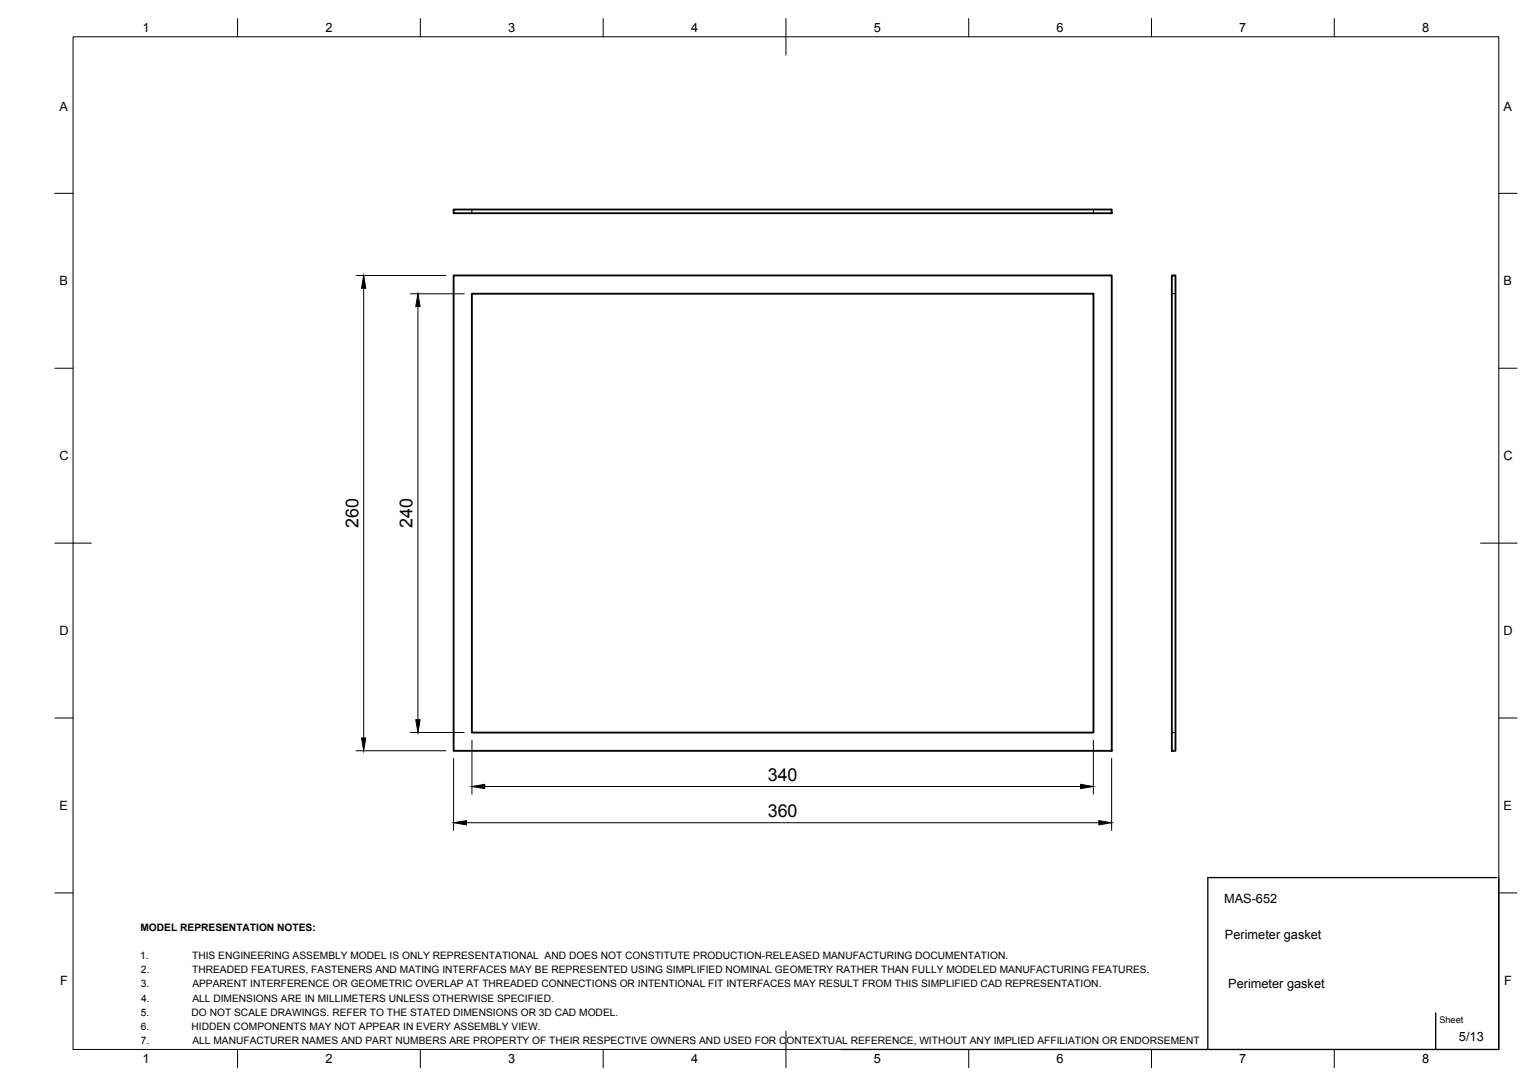
ISO-10303-21;
HEADER;
/* Generated by software containing ST-Developer
 * from STEP Tools, Inc. (www.steptools.com) 
 */

FILE_DESCRIPTION(
/* description */ ('Independent hinged machine back cover with retained hinge pins, perim
eter gasket and quarter-turn cam latch. Nominal cover 360 x 260 x 3 mm
, frame 430 x 300 x 20 mm. No guarding, structural or ingress rating a
ssigned.'),
/* implementation_level */ '2;1');

FILE_NAME(
/* name */ 'Perimeter gasket.step',
/* time_stamp */ '2026-11-09T19:36:59-08:00',
/* author */ (''),
/* organization */ (''),
/* preprocessor_version */ 'ST-DEVELOPER v20.2',
/* originating_system */ 'Autodesk Translation Framework v15.17.0.0',
/* authorisation */ '');

FILE_SCHEMA (('AUTOMOTIVE_DESIGN { 1 0 10303 214 3 1 1 }'));
ENDSEC;

DATA;
#10=MECHANICAL_DESIGN_GEOMETRIC_PRESENTATION_REPRESENTATION('',(#200),#32627);
#164=SHAPE_REPRESENTATION_RELATIONSHIP('SRR','None',#32710,#182);
#182=ADVANCED_BREP_SHAPE_REPRESENTATION('',(#218),#32611);
#200=STYLED_ITEM('',(#32809),#218);
#218=MANIFOLD_SOLID_BREP('Body1',#8677);
#250=FACE_BOUND('',#1133,.T.);
#251=FACE_BOUND('',#1135,.T.);
#335=PLANE('',#9103);
#336=PLANE('',#9104);
#337=PLANE('',#9105);
#338=PLANE('',#9106);
#339=PLANE('',#9107);
#340=PLANE('',#9108);
#341=PLANE('',#9109);
#342=PLANE('',#9110);
#343=PLANE('',#9111);
#344=PLANE('',#9112);
#633=FACE_OUTER_BOUND('',#1124,.T.);
#634=FACE_OUTER_BOUND('',#1125,.T.);
#635=FACE_OUTER_BOUND('',#1126,.T.);
#636=FACE_OUTER_BOUND('',#1127,.T.);
#637=FACE_OUTER_BOUND('',#1128,.T.);
#638=FACE_OUTER_BOUND('',#1129,.T.);
#639=FACE_OUTER_BOUND('',#1130,.T.);
#640=FACE_OUTER_BOUND('',#1131,.T.);
#641=FACE_OUTER_BOUND('',#1132,.T.);
#642=FACE_OUTER_BOUND('',#1134,.T.);
#1124=EDGE_LOOP('',(#6405,#6406,#6407,#6408));
#1125=EDGE_LOOP('',(#6409,#6410,#6411,#6412));
#1126=EDGE_LOOP('',(#6413,#6414,#6415,#6416));
#1127=EDGE_LOOP('',(#6417,#6418,#6419,#6420));
#1128=EDGE_LOOP('',(#6421,#6422,#6423,#6424));
#1129=EDGE_LOOP('',(#6425,#6426,#6427,#6428));
#1130=EDGE_LOOP('',(#6429,#6430,#6431,#6432));
#1131=EDGE_LOOP('',(#6433,#6434,#6435,#6436));
#1132=EDGE_LOOP('',(#6437,#6438,#6439,#6440));
#1133=EDGE_LOOP('',(#6441,#6442,#6443,#6444));
#1134=EDGE_LOOP('',(#6445,#6446,#6447,#6448));
#1135=EDGE_LOOP('',(#6449,#6450,#6451,#6452));
#2356=LINE('',#21698,#2902);
#2357=LINE('',#21700,#2903);
#2358=LINE('',#21702,#2904);
#2359=LINE('',#21703,#2905);
#2360=LINE('',#21706,#2906);
#2361=LINE('',#21708,#2907);
#2362=LINE('',#21709,#2908);
#2363=LINE('',#21712,#2909);
#2364=LINE('',#21714,#2910);
#2365=LINE('',#21715,#2911);
#2366=LINE('',#21717,#2912);
#2367=LINE('',#21718,#2913);
#2368=LINE('',#21722,#2914);
#2369=LINE('',#21724,#2915);
#2370=LINE('',#21726,#2916);
#2371=LINE('',#21727,#2917);
#2372=LINE('',#21730,#2918);
#2373=LINE('',#21732,#2919);
#2374=LINE('',#21733,#2920);
#2375=LINE('',#21736,#2921);
#2376=LINE('',#21738,#2922);
#2377=LINE('',#21739,#2923);
#2378=LINE('',#21741,#2924);
#2379=LINE('',#21742,#2925);
#2902=VECTOR('',#10134,10.);
#2903=VECTOR('',#10135,10.);
#2904=VECTOR('',#10136,10.);
#2905=VECTOR('',#10137,10.);
#2906=VECTOR('',#10140,10.);
#2907=VECTOR('',#10141,10.);
#2908=VECTOR('',#10142,10.);
#2909=VECTOR('',#10145,10.);
#2910=VECTOR('',#10146,10.);
#2911=VECTOR('',#10147,10.);
#2912=VECTOR('',#10150,10.);
#2913=VECTOR('',#10151,10.);
#2914=VECTOR('',#10154,10.);
#2915=VECTOR('',#10155,10.);
#2916=VECTOR('',#10156,10.);
#2917=VECTOR('',#10157,10.);
#2918=VECTOR('',#10160,10.);
#2919=VECTOR('',#10161,10.);
#2920=VECTOR('',#10162,10.);
#2921=VECTOR('',#10165,10.);
#2922=VECTOR('',#10166,10.);
#2923=VECTOR('',#10167,10.);
#2924=VECTOR('',#10170,10.);
#2925=VECTOR('',#10171,10.);
#3613=VERTEX_POINT('',#21696);
#3614=VERTEX_POINT('',#21697);
#3615=VERTEX_POINT('',#21699);
#3616=VERTEX_POINT('',#21701);
#3617=VERTEX_POINT('',#21705);
#3618=VERTEX_POINT('',#21707);
#3619=VERTEX_POINT('',#21711);
#3620=VERTEX_POINT('',#21713);
#3621=VERTEX_POINT('',#21720);
#3622=VERTEX_POINT('',#21721);
#3623=VERTEX_POINT('',#21723);
#3624=VERTEX_POINT('',#21725);
#3625=VERTEX_POINT('',#21729);
#3626=VERTEX_POINT('',#21731);
#3627=VERTEX_POINT('',#21735);
#3628=VERTEX_POINT('',#21737);
#4626=EDGE_CURVE('',#3613,#3614,#2356,.T.);
#4627=EDGE_CURVE('',#3614,#3615,#2357,.T.);
#4628=EDGE_CURVE('',#3616,#3615,#2358,.T.);
#4629=EDGE_CURVE('',#3613,#3616,#2359,.T.);
#4630=EDGE_CURVE('',#3617,#3613,#2360,.T.);
#4631=EDGE_CURVE('',#3618,#3616,#2361,.T.);
#4632=EDGE_CURVE('',#3617,#3618,#2362,.T.);
#4633=EDGE_CURVE('',#3619,#3617,#2363,.T.);
#4634=EDGE_CURVE('',#3620,#3618,#2364,.T.);
#4635=EDGE_CURVE('',#3619,#3620,#2365,.T.);
#4636=EDGE_CURVE('',#3614,#3619,#2366,.T.);
#4637=EDGE_CURVE('',#3615,#3620,#2367,.T.);
#4638=EDGE_CURVE('',#3621,#3622,#2368,.T.);
#4639=EDGE_CURVE('',#3622,#3623,#2369,.T.);
#4640=EDGE_CURVE('',#3624,#3623,#2370,.T.);
#4641=EDGE_CURVE('',#3621,#3624,#2371,.T.);
#4642=EDGE_CURVE('',#3625,#3621,#2372,.T.);
#4643=EDGE_CURVE('',#3626,#3624,#2373,.T.);
#4644=EDGE_CURVE('',#3625,#3626,#2374,.T.);
#4645=EDGE_CURVE('',#3627,#3625,#2375,.T.);
#4646=EDGE_CURVE('',#3628,#3626,#2376,.T.);
#4647=EDGE_CURVE('',#3627,#3628,#2377,.T.);
#4648=EDGE_CURVE('',#3622,#3627,#2378,.T.);
#4649=EDGE_CURVE('',#3623,#3628,#2379,.T.);
#6405=ORIENTED_EDGE('',*,*,#4626,.T.);
#6406=ORIENTED_EDGE('',*,*,#4627,.T.);
#6407=ORIENTED_EDGE('',*,*,#4628,.F.);
#6408=ORIENTED_EDGE('',*,*,#4629,.F.);
#6409=ORIENTED_EDGE('',*,*,#4630,.T.);
#6410=ORIENTED_EDGE('',*,*,#4629,.T.);
#6411=ORIENTED_EDGE('',*,*,#4631,.F.);
#6412=ORIENTED_EDGE('',*,*,#4632,.F.);
#6413=ORIENTED_EDGE('',*,*,#4633,.T.);
#6414=ORIENTED_EDGE('',*,*,#4632,.T.);
#6415=ORIENTED_EDGE('',*,*,#4634,.F.);
#6416=ORIENTED_EDGE('',*,*,#4635,.F.);
#6417=ORIENTED_EDGE('',*,*,#4636,.T.);
#6418=ORIENTED_EDGE('',*,*,#4635,.T.);
#6419=ORIENTED_EDGE('',*,*,#4637,.F.);
#6420=ORIENTED_EDGE('',*,*,#4627,.F.);
#6421=ORIENTED_EDGE('',*,*,#4638,.T.);
#6422=ORIENTED_EDGE('',*,*,#4639,.T.);
#6423=ORIENTED_EDGE('',*,*,#4640,.F.);
#6424=ORIENTED_EDGE('',*,*,#4641,.F.);
#6425=ORIENTED_EDGE('',*,*,#4642,.T.);
#6426=ORIENTED_EDGE('',*,*,#4641,.T.);
#6427=ORIENTED_EDGE('',*,*,#4643,.F.);
#6428=ORIENTED_EDGE('',*,*,#4644,.F.);
#6429=ORIENTED_EDGE('',*,*,#4645,.T.);
#6430=ORIENTED_EDGE('',*,*,#4644,.T.);
#6431=ORIENTED_EDGE('',*,*,#4646,.F.);
#6432=ORIENTED_EDGE('',*,*,#4647,.F.);
#6433=ORIENTED_EDGE('',*,*,#4648,.T.);
#6434=ORIENTED_EDGE('',*,*,#4647,.T.);
#6435=ORIENTED_EDGE('',*,*,#4649,.F.);
#6436=ORIENTED_EDGE('',*,*,#4639,.F.);
#6437=ORIENTED_EDGE('',*,*,#4649,.T.);
#6438=ORIENTED_EDGE('',*,*,#4646,.T.);
#6439=ORIENTED_EDGE('',*,*,#4643,.T.);
#6440=ORIENTED_EDGE('',*,*,#4640,.T.);
#6441=ORIENTED_EDGE('',*,*,#4637,.T.);
#6442=ORIENTED_EDGE('',*,*,#4634,.T.);
#6443=ORIENTED_EDGE('',*,*,#4631,.T.);
#6444=ORIENTED_EDGE('',*,*,#4628,.T.);
#6445=ORIENTED_EDGE('',*,*,#4648,.F.);
#6446=ORIENTED_EDGE('',*,*,#4638,.F.);
#6447=ORIENTED_EDGE('',*,*,#4642,.F.);
#6448=ORIENTED_EDGE('',*,*,#4645,.F.);
#6449=ORIENTED_EDGE('',*,*,#4636,.F.);
#6450=ORIENTED_EDGE('',*,*,#4626,.F.);
#6451=ORIENTED_EDGE('',*,*,#4630,.F.);
#6452=ORIENTED_EDGE('',*,*,#4633,.F.);
#8381=ADVANCED_FACE('',(#633),#335,.T.);
#8382=ADVANCED_FACE('',(#634),#336,.T.);
#8383=ADVANCED_FACE('',(#635),#337,.T.);
#8384=ADVANCED_FACE('',(#636),#338,.T.);
#8385=ADVANCED_FACE('',(#637),#339,.T.);
#8386=ADVANCED_FACE('',(#638),#340,.T.);
#8387=ADVANCED_FACE('',(#639),#341,.T.);
#8388=ADVANCED_FACE('',(#640),#342,.T.);
#8389=ADVANCED_FACE('',(#641,#250),#343,.T.);
#8390=ADVANCED_FACE('',(#642,#251),#344,.F.);
#8677=CLOSED_SHELL('',(#8381,#8382,#8383,#8384,#8385,#8386,#8387,#8388,
#8389,#8390));
#9102=AXIS2_PLACEMENT_3D('',#21694,#10130,#10131);
#9103=AXIS2_PLACEMENT_3D('',#21695,#10132,#10133);
#9104=AXIS2_PLACEMENT_3D('',#21704,#10138,#10139);
#9105=AXIS2_PLACEMENT_3D('',#21710,#10143,#10144);
#9106=AXIS2_PLACEMENT_3D('',#21716,#10148,#10149);
#9107=AXIS2_PLACEMENT_3D('',#21719,#10152,#10153);
#9108=AXIS2_PLACEMENT_3D('',#21728,#10158,#10159);
#9109=AXIS2_PLACEMENT_3D('',#21734,#10163,#10164);
#9110=AXIS2_PLACEMENT_3D('',#21740,#10168,#10169);
#9111=AXIS2_PLACEMENT_3D('',#21743,#10172,#10173);
#9112=AXIS2_PLACEMENT_3D('',#21744,#10174,#10175);
#10130=DIRECTION('axis',(0.,0.,1.));
#10131=DIRECTION('refdir',(1.,0.,0.));
#10132=DIRECTION('center_axis',(0.,1.,0.));
#10133=DIRECTION('ref_axis',(-1.,0.,0.));
#10134=DIRECTION('',(-1.,0.,0.));
#10135=DIRECTION('',(0.,0.,1.));
#10136=DIRECTION('',(-1.,0.,0.));
#10137=DIRECTION('',(0.,0.,1.));
#10138=DIRECTION('center_axis',(-1.,0.,0.));
#10139=DIRECTION('ref_axis',(0.,-1.,0.));
#10140=DIRECTION('',(0.,-1.,0.));
#10141=DIRECTION('',(0.,-1.,0.));
#10142=DIRECTION('',(0.,0.,1.));
#10143=DIRECTION('center_axis',(0.,-1.,0.));
#10144=DIRECTION('ref_axis',(1.,0.,0.));
#10145=DIRECTION('',(1.,0.,0.));
#10146=DIRECTION('',(1.,0.,0.));
#10147=DIRECTION('',(0.,0.,1.));
#10148=DIRECTION('center_axis',(1.,0.,0.));
#10149=DIRECTION('ref_axis',(0.,1.,0.));
#10150=DIRECTION('',(0.,1.,0.));
#10151=DIRECTION('',(0.,1.,0.));
#10152=DIRECTION('center_axis',(0.,1.,0.));
#10153=DIRECTION('ref_axis',(-1.,0.,0.));
#10154=DIRECTION('',(-1.,0.,0.));
#10155=DIRECTION('',(0.,0.,1.));
#10156=DIRECTION('',(-1.,0.,0.));
#10157=DIRECTION('',(0.,0.,1.));
#10158=DIRECTION('center_axis',(1.,0.,0.));
#10159=DIRECTION('ref_axis',(0.,1.,0.));
#10160=DIRECTION('',(0.,1.,0.));
#10161=DIRECTION('',(0.,1.,0.));
#10162=DIRECTION('',(0.,0.,1.));
#10163=DIRECTION('center_axis',(0.,-1.,0.));
#10164=DIRECTION('ref_axis',(1.,0.,0.));
#10165=DIRECTION('',(1.,0.,0.));
#10166=DIRECTION('',(1.,0.,0.));
#10167=DIRECTION('',(0.,0.,1.));
#10168=DIRECTION('center_axis',(-1.,0.,0.));
#10169=DIRECTION('ref_axis',(0.,-1.,0.));
#10170=DIRECTION('',(0.,-1.,0.));
#10171=DIRECTION('',(0.,-1.,0.));
#10172=DIRECTION('center_axis',(0.,0.,1.));
#10173=DIRECTION('ref_axis',(1.,0.,0.));
#10174=DIRECTION('center_axis',(0.,0.,1.));
#10175=DIRECTION('ref_axis',(1.,0.,0.));
#21694=CARTESIAN_POINT('',(0.,0.,0.));
#21695=CARTESIAN_POINT('Origin',(170.,-120.,0.));
#21696=CARTESIAN_POINT('',(170.,-120.,0.));
#21697=CARTESIAN_POINT('',(-170.,-120.,0.));
#21698=CARTESIAN_POINT('',(-170.,-120.,0.));
#21699=CARTESIAN_POINT('',(-170.,-120.,2.));
#21700=CARTESIAN_POINT('',(-170.,-120.,0.));
#21701=CARTESIAN_POINT('',(170.,-120.,2.));
#21702=CARTESIAN_POINT('',(-170.,-120.,2.));
#21703=CARTESIAN_POINT('',(170.,-120.,0.));
#21704=CARTESIAN_POINT('Origin',(170.,120.,0.));
#21705=CARTESIAN_POINT('',(170.,120.,0.));
#21706=CARTESIAN_POINT('',(170.,-120.,0.));
#21707=CARTESIAN_POINT('',(170.,120.,2.));
#21708=CARTESIAN_POINT('',(170.,-120.,2.));
#21709=CARTESIAN_POINT('',(170.,120.,0.));
#21710=CARTESIAN_POINT('Origin',(-170.,120.,0.));
#21711=CARTESIAN_POINT('',(-170.,120.,0.));
#21712=CARTESIAN_POINT('',(170.,120.,0.));
#21713=CARTESIAN_POINT('',(-170.,120.,2.));
#21714=CARTESIAN_POINT('',(170.,120.,2.));
#21715=CARTESIAN_POINT('',(-170.,120.,0.));
#21716=CARTESIAN_POINT('Origin',(-170.,-120.,0.));
#21717=CARTESIAN_POINT('',(-170.,120.,0.));
#21718=CARTESIAN_POINT('',(-170.,120.,2.));
#21719=CARTESIAN_POINT('Origin',(180.,130.,0.));
#21720=CARTESIAN_POINT('',(180.,130.,0.));
#21721=CARTESIAN_POINT('',(-180.,130.,0.));
#21722=CARTESIAN_POINT('',(180.,130.,0.));
#21723=CARTESIAN_POINT('',(-180.,130.,2.));
#21724=CARTESIAN_POINT('',(-180.,130.,0.));
#21725=CARTESIAN_POINT('',(180.,130.,2.));
#21726=CARTESIAN_POINT('',(180.,130.,2.));
#21727=CARTESIAN_POINT('',(180.,130.,0.));
#21728=CARTESIAN_POINT('Origin',(180.,-130.,0.));
#21729=CARTESIAN_POINT('',(180.,-130.,0.));
#21730=CARTESIAN_POINT('',(180.,-130.,0.));
#21731=CARTESIAN_POINT('',(180.,-130.,2.));
#21732=CARTESIAN_POINT('',(180.,-130.,2.));
#21733=CARTESIAN_POINT('',(180.,-130.,0.));
#21734=CARTESIAN_POINT('Origin',(-180.,-130.,0.));
#21735=CARTESIAN_POINT('',(-180.,-130.,0.));
#21736=CARTESIAN_POINT('',(-180.,-130.,0.));
#21737=CARTESIAN_POINT('',(-180.,-130.,2.));
#21738=CARTESIAN_POINT('',(-180.,-130.,2.));
#21739=CARTESIAN_POINT('',(-180.,-130.,0.));
#21740=CARTESIAN_POINT('Origin',(-180.,130.,0.));
#21741=CARTESIAN_POINT('',(-180.,130.,0.));
#21742=CARTESIAN_POINT('',(-180.,130.,2.));
#21743=CARTESIAN_POINT('Origin',(0.,0.,2.));
#21744=CARTESIAN_POINT('Origin',(0.,0.,0.));
#32591=UNCERTAINTY_MEASURE_WITH_UNIT(LENGTH_MEASURE(0.01),#32628,
'DISTANCE_ACCURACY_VALUE',
'Maximum model space distance between geometric entities at asserted c
onnectivities');
#32607=UNCERTAINTY_MEASURE_WITH_UNIT(LENGTH_MEASURE(0.01),#32628,
'DISTANCE_ACCURACY_VALUE',
'Maximum model space distance between geometric entities at asserted c
onnectivities');
#32611=(
GEOMETRIC_REPRESENTATION_CONTEXT(3)
GLOBAL_UNCERTAINTY_ASSIGNED_CONTEXT((#32591))
GLOBAL_UNIT_ASSIGNED_CONTEXT((#32628,#32630,#32631))
REPRESENTATION_CONTEXT('','3D')
);
#32627=(
GEOMETRIC_REPRESENTATION_CONTEXT(3)
GLOBAL_UNCERTAINTY_ASSIGNED_CONTEXT((#32607))
GLOBAL_UNIT_ASSIGNED_CONTEXT((#32628,#32630,#32631))
REPRESENTATION_CONTEXT('','3D')
);
#32628=(
LENGTH_UNIT()
NAMED_UNIT(*)
SI_UNIT(.MILLI.,.METRE.)
);
#32630=(
NAMED_UNIT(*)
PLANE_ANGLE_UNIT()
SI_UNIT($,.RADIAN.)
);
#32631=(
NAMED_UNIT(*)
SI_UNIT($,.STERADIAN.)
SOLID_ANGLE_UNIT()
);
#32635=SHAPE_DEFINITION_REPRESENTATION(#32654,#32710);
#32654=PRODUCT_DEFINITION_SHAPE('',$,#32730);
#32710=SHAPE_REPRESENTATION('',(#9102),#32611);
#32726=PRODUCT_DEFINITION_CONTEXT('part definition',#32785,'design');
#32730=PRODUCT_DEFINITION('Perimeter gasket','Perimeter gasket',#32749,
#32726);
#32749=PRODUCT_DEFINITION_FORMATION('',$,#32790);
#32785=APPLICATION_CONTEXT(
'Core Data for Automotive Mechanical Design Process');
#32786=PRODUCT_CONTEXT('part definition',#32785,'mechanical');
#32790=PRODUCT('Perimeter gasket','Perimeter gasket',$,(#32786));
#32809=PRESENTATION_STYLE_ASSIGNMENT((#32816));
#32816=SURFACE_STYLE_USAGE(.BOTH.,#32823);
#32823=SURFACE_SIDE_STYLE('',(#32830));
#32830=SURFACE_STYLE_FILL_AREA(#32837);
#32837=FILL_AREA_STYLE('Dark gray',(#32844));
#32844=FILL_AREA_STYLE_COLOUR('Dark gray',#32851);
#32851=COLOUR_RGB('Dark gray',0.250980392156863,0.282352941176471,0.32156862745098);
ENDSEC;
END-ISO-10303-21;
